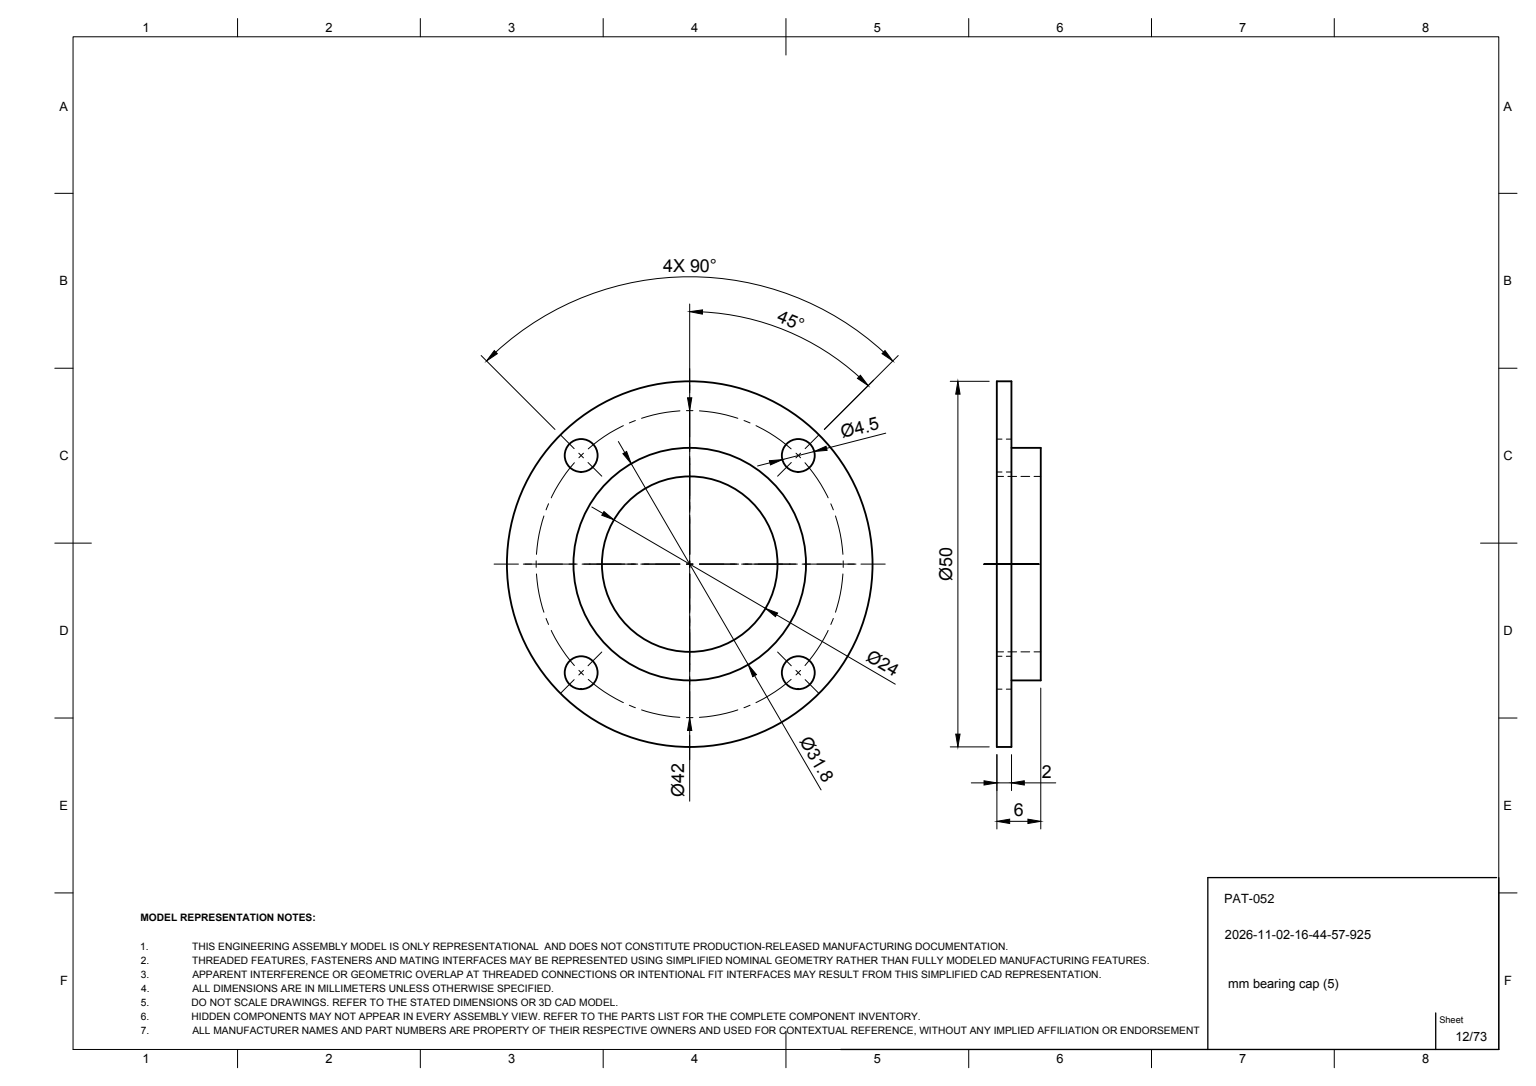
ISO-10303-21;
HEADER;
/* Generated by software containing ST-Developer
 * from STEP Tools, Inc. (www.steptools.com) 
 */

FILE_DESCRIPTION(
/* description */ ('Hand-crank gear train demonstrator'),
/* implementation_level */ '2;1');

FILE_NAME(
/* name */ 'mm bearing cap (5).step',
/* time_stamp */ '2026-10-28T03:22:13-07:00',
/* author */ (''),
/* organization */ (''),
/* preprocessor_version */ 'ST-DEVELOPER v20.2',
/* originating_system */ 'Autodesk Translation Framework v15.17.0.0',
/* authorisation */ '');

FILE_SCHEMA (('AUTOMOTIVE_DESIGN { 1 0 10303 214 3 1 1 }'));
ENDSEC;

DATA;
#10=MECHANICAL_DESIGN_GEOMETRIC_PRESENTATION_REPRESENTATION('',(#1197),#62758);
#1069=SHAPE_REPRESENTATION_RELATIONSHIP('SRR','None',#63041,#1133);
#1133=ADVANCED_BREP_SHAPE_REPRESENTATION('',(#1275),#62695);
#1197=STYLED_ITEM('',(#63462),#1275);
#1275=MANIFOLD_SOLID_BREP('Body1',#16378);
#1454=FACE_BOUND('',#3285,.T.);
#1455=FACE_BOUND('',#3289,.T.);
#1456=FACE_BOUND('',#3290,.T.);
#1457=FACE_BOUND('',#3291,.T.);
#1458=FACE_BOUND('',#3292,.T.);
#1459=FACE_BOUND('',#3293,.T.);
#1460=FACE_BOUND('',#3295,.T.);
#1461=FACE_BOUND('',#3296,.T.);
#1462=FACE_BOUND('',#3297,.T.);
#1463=FACE_BOUND('',#3298,.T.);
#1464=FACE_BOUND('',#3299,.T.);
#1673=PLANE('',#17425);
#1674=PLANE('',#17432);
#1675=PLANE('',#17433);
#2231=FACE_OUTER_BOUND('',#3279,.T.);
#2232=FACE_OUTER_BOUND('',#3280,.T.);
#2233=FACE_OUTER_BOUND('',#3281,.T.);
#2234=FACE_OUTER_BOUND('',#3282,.T.);
#2235=FACE_OUTER_BOUND('',#3283,.T.);
#2236=FACE_OUTER_BOUND('',#3284,.T.);
#2237=FACE_OUTER_BOUND('',#3286,.T.);
#2238=FACE_OUTER_BOUND('',#3287,.T.);
#2239=FACE_OUTER_BOUND('',#3288,.T.);
#2240=FACE_OUTER_BOUND('',#3294,.T.);
#3279=EDGE_LOOP('',(#11333,#11334,#11335,#11336));
#3280=EDGE_LOOP('',(#11337,#11338,#11339,#11340));
#3281=EDGE_LOOP('',(#11341,#11342,#11343,#11344));
#3282=EDGE_LOOP('',(#11345,#11346,#11347,#11348));
#3283=EDGE_LOOP('',(#11349,#11350,#11351,#11352));
#3284=EDGE_LOOP('',(#11353));
#3285=EDGE_LOOP('',(#11354));
#3286=EDGE_LOOP('',(#11355,#11356,#11357,#11358));
#3287=EDGE_LOOP('',(#11359,#11360,#11361,#11362));
#3288=EDGE_LOOP('',(#11363));
#3289=EDGE_LOOP('',(#11364));
#3290=EDGE_LOOP('',(#11365));
#3291=EDGE_LOOP('',(#11366));
#3292=EDGE_LOOP('',(#11367));
#3293=EDGE_LOOP('',(#11368));
#3294=EDGE_LOOP('',(#11369));
#3295=EDGE_LOOP('',(#11370));
#3296=EDGE_LOOP('',(#11371));
#3297=EDGE_LOOP('',(#11372));
#3298=EDGE_LOOP('',(#11373));
#3299=EDGE_LOOP('',(#11374));
#4402=LINE('',#23846,#5534);
#4403=LINE('',#23852,#5535);
#4404=LINE('',#23858,#5536);
#4405=LINE('',#23864,#5537);
#4406=LINE('',#23870,#5538);
#4407=LINE('',#23878,#5539);
#4408=LINE('',#23883,#5540);
#5534=VECTOR('',#19455,0.225);
#5535=VECTOR('',#19462,0.225);
#5536=VECTOR('',#19469,0.225);
#5537=VECTOR('',#19476,0.225);
#5538=VECTOR('',#19483,1.59);
#5539=VECTOR('',#19494,1.2);
#5540=VECTOR('',#19499,2.5);
#6683=CIRCLE('',#17411,0.225);
#6684=CIRCLE('',#17412,0.225);
#6685=CIRCLE('',#17414,0.225);
#6686=CIRCLE('',#17415,0.225);
#6687=CIRCLE('',#17417,0.225);
#6688=CIRCLE('',#17418,0.225);
#6689=CIRCLE('',#17420,0.225);
#6690=CIRCLE('',#17421,0.225);
#6691=CIRCLE('',#17423,1.59);
#6692=CIRCLE('',#17424,1.59);
#6693=CIRCLE('',#17426,1.2);
#6694=CIRCLE('',#17428,1.2);
#6695=CIRCLE('',#17430,2.5);
#6696=CIRCLE('',#17431,2.5);
#7377=VERTEX_POINT('',#23843);
#7378=VERTEX_POINT('',#23845);
#7379=VERTEX_POINT('',#23849);
#7380=VERTEX_POINT('',#23851);
#7381=VERTEX_POINT('',#23855);
#7382=VERTEX_POINT('',#23857);
#7383=VERTEX_POINT('',#23861);
#7384=VERTEX_POINT('',#23863);
#7385=VERTEX_POINT('',#23867);
#7386=VERTEX_POINT('',#23869);
#7387=VERTEX_POINT('',#23873);
#7388=VERTEX_POINT('',#23876);
#7389=VERTEX_POINT('',#23880);
#7390=VERTEX_POINT('',#23882);
#8918=EDGE_CURVE('',#7377,#7377,#6683,.T.);
#8919=EDGE_CURVE('',#7377,#7378,#4402,.T.);
#8920=EDGE_CURVE('',#7378,#7378,#6684,.T.);
#8921=EDGE_CURVE('',#7379,#7379,#6685,.T.);
#8922=EDGE_CURVE('',#7379,#7380,#4403,.T.);
#8923=EDGE_CURVE('',#7380,#7380,#6686,.T.);
#8924=EDGE_CURVE('',#7381,#7381,#6687,.T.);
#8925=EDGE_CURVE('',#7381,#7382,#4404,.T.);
#8926=EDGE_CURVE('',#7382,#7382,#6688,.T.);
#8927=EDGE_CURVE('',#7383,#7383,#6689,.T.);
#8928=EDGE_CURVE('',#7383,#7384,#4405,.T.);
#8929=EDGE_CURVE('',#7384,#7384,#6690,.T.);
#8930=EDGE_CURVE('',#7385,#7385,#6691,.T.);
#8931=EDGE_CURVE('',#7385,#7386,#4406,.T.);
#8932=EDGE_CURVE('',#7386,#7386,#6692,.T.);
#8933=EDGE_CURVE('',#7387,#7387,#6693,.T.);
#8934=EDGE_CURVE('',#7388,#7388,#6694,.T.);
#8935=EDGE_CURVE('',#7388,#7387,#4407,.T.);
#8936=EDGE_CURVE('',#7389,#7389,#6695,.T.);
#8937=EDGE_CURVE('',#7389,#7390,#4408,.T.);
#8938=EDGE_CURVE('',#7390,#7390,#6696,.T.);
#11333=ORIENTED_EDGE('',*,*,#8918,.F.);
#11334=ORIENTED_EDGE('',*,*,#8919,.T.);
#11335=ORIENTED_EDGE('',*,*,#8920,.F.);
#11336=ORIENTED_EDGE('',*,*,#8919,.F.);
#11337=ORIENTED_EDGE('',*,*,#8921,.F.);
#11338=ORIENTED_EDGE('',*,*,#8922,.T.);
#11339=ORIENTED_EDGE('',*,*,#8923,.F.);
#11340=ORIENTED_EDGE('',*,*,#8922,.F.);
#11341=ORIENTED_EDGE('',*,*,#8924,.F.);
#11342=ORIENTED_EDGE('',*,*,#8925,.T.);
#11343=ORIENTED_EDGE('',*,*,#8926,.F.);
#11344=ORIENTED_EDGE('',*,*,#8925,.F.);
#11345=ORIENTED_EDGE('',*,*,#8927,.F.);
#11346=ORIENTED_EDGE('',*,*,#8928,.T.);
#11347=ORIENTED_EDGE('',*,*,#8929,.F.);
#11348=ORIENTED_EDGE('',*,*,#8928,.F.);
#11349=ORIENTED_EDGE('',*,*,#8930,.F.);
#11350=ORIENTED_EDGE('',*,*,#8931,.T.);
#11351=ORIENTED_EDGE('',*,*,#8932,.T.);
#11352=ORIENTED_EDGE('',*,*,#8931,.F.);
#11353=ORIENTED_EDGE('',*,*,#8932,.F.);
#11354=ORIENTED_EDGE('',*,*,#8933,.F.);
#11355=ORIENTED_EDGE('',*,*,#8934,.F.);
#11356=ORIENTED_EDGE('',*,*,#8935,.T.);
#11357=ORIENTED_EDGE('',*,*,#8933,.T.);
#11358=ORIENTED_EDGE('',*,*,#8935,.F.);
#11359=ORIENTED_EDGE('',*,*,#8936,.F.);
#11360=ORIENTED_EDGE('',*,*,#8937,.T.);
#11361=ORIENTED_EDGE('',*,*,#8938,.T.);
#11362=ORIENTED_EDGE('',*,*,#8937,.F.);
#11363=ORIENTED_EDGE('',*,*,#8936,.T.);
#11364=ORIENTED_EDGE('',*,*,#8934,.T.);
#11365=ORIENTED_EDGE('',*,*,#8929,.T.);
#11366=ORIENTED_EDGE('',*,*,#8926,.T.);
#11367=ORIENTED_EDGE('',*,*,#8923,.T.);
#11368=ORIENTED_EDGE('',*,*,#8920,.T.);
#11369=ORIENTED_EDGE('',*,*,#8938,.F.);
#11370=ORIENTED_EDGE('',*,*,#8930,.T.);
#11371=ORIENTED_EDGE('',*,*,#8927,.T.);
#11372=ORIENTED_EDGE('',*,*,#8924,.T.);
#11373=ORIENTED_EDGE('',*,*,#8921,.T.);
#11374=ORIENTED_EDGE('',*,*,#8918,.T.);
#15232=CYLINDRICAL_SURFACE('',#17410,0.225);
#15233=CYLINDRICAL_SURFACE('',#17413,0.225);
#15234=CYLINDRICAL_SURFACE('',#17416,0.225);
#15235=CYLINDRICAL_SURFACE('',#17419,0.225);
#15236=CYLINDRICAL_SURFACE('',#17422,1.59);
#15237=CYLINDRICAL_SURFACE('',#17427,1.2);
#15238=CYLINDRICAL_SURFACE('',#17429,2.5);
#15541=ADVANCED_FACE('',(#2231),#15232,.F.);
#15542=ADVANCED_FACE('',(#2232),#15233,.F.);
#15543=ADVANCED_FACE('',(#2233),#15234,.F.);
#15544=ADVANCED_FACE('',(#2234),#15235,.F.);
#15545=ADVANCED_FACE('',(#2235),#15236,.T.);
#15546=ADVANCED_FACE('',(#2236,#1454),#1673,.F.);
#15547=ADVANCED_FACE('',(#2237),#15237,.F.);
#15548=ADVANCED_FACE('',(#2238),#15238,.T.);
#15549=ADVANCED_FACE('',(#2239,#1455,#1456,#1457,#1458,#1459),#1674,.T.);
#15550=ADVANCED_FACE('',(#2240,#1460,#1461,#1462,#1463,#1464),#1675,.F.);
#16378=CLOSED_SHELL('',(#15541,#15542,#15543,#15544,#15545,#15546,#15547,
#15548,#15549,#15550));
#17409=AXIS2_PLACEMENT_3D('',#23841,#19449,#19450);
#17410=AXIS2_PLACEMENT_3D('',#23842,#19451,#19452);
#17411=AXIS2_PLACEMENT_3D('',#23844,#19453,#19454);
#17412=AXIS2_PLACEMENT_3D('',#23847,#19456,#19457);
#17413=AXIS2_PLACEMENT_3D('',#23848,#19458,#19459);
#17414=AXIS2_PLACEMENT_3D('',#23850,#19460,#19461);
#17415=AXIS2_PLACEMENT_3D('',#23853,#19463,#19464);
#17416=AXIS2_PLACEMENT_3D('',#23854,#19465,#19466);
#17417=AXIS2_PLACEMENT_3D('',#23856,#19467,#19468);
#17418=AXIS2_PLACEMENT_3D('',#23859,#19470,#19471);
#17419=AXIS2_PLACEMENT_3D('',#23860,#19472,#19473);
#17420=AXIS2_PLACEMENT_3D('',#23862,#19474,#19475);
#17421=AXIS2_PLACEMENT_3D('',#23865,#19477,#19478);
#17422=AXIS2_PLACEMENT_3D('',#23866,#19479,#19480);
#17423=AXIS2_PLACEMENT_3D('',#23868,#19481,#19482);
#17424=AXIS2_PLACEMENT_3D('',#23871,#19484,#19485);
#17425=AXIS2_PLACEMENT_3D('',#23872,#19486,#19487);
#17426=AXIS2_PLACEMENT_3D('',#23874,#19488,#19489);
#17427=AXIS2_PLACEMENT_3D('',#23875,#19490,#19491);
#17428=AXIS2_PLACEMENT_3D('',#23877,#19492,#19493);
#17429=AXIS2_PLACEMENT_3D('',#23879,#19495,#19496);
#17430=AXIS2_PLACEMENT_3D('',#23881,#19497,#19498);
#17431=AXIS2_PLACEMENT_3D('',#23884,#19500,#19501);
#17432=AXIS2_PLACEMENT_3D('',#23885,#19502,#19503);
#17433=AXIS2_PLACEMENT_3D('',#23886,#19504,#19505);
#19449=DIRECTION('axis',(0.,0.,1.));
#19450=DIRECTION('refdir',(1.,0.,0.));
#19451=DIRECTION('center_axis',(0.,1.,0.));
#19452=DIRECTION('ref_axis',(1.,0.,0.));
#19453=DIRECTION('center_axis',(0.,1.,0.));
#19454=DIRECTION('ref_axis',(1.,0.,0.));
#19455=DIRECTION('',(0.,1.,0.));
#19456=DIRECTION('center_axis',(0.,-1.,0.));
#19457=DIRECTION('ref_axis',(1.,0.,0.));
#19458=DIRECTION('center_axis',(0.,1.,0.));
#19459=DIRECTION('ref_axis',(1.,0.,0.));
#19460=DIRECTION('center_axis',(0.,1.,0.));
#19461=DIRECTION('ref_axis',(1.,0.,0.));
#19462=DIRECTION('',(0.,1.,0.));
#19463=DIRECTION('center_axis',(0.,-1.,0.));
#19464=DIRECTION('ref_axis',(1.,0.,0.));
#19465=DIRECTION('center_axis',(0.,1.,0.));
#19466=DIRECTION('ref_axis',(1.,0.,0.));
#19467=DIRECTION('center_axis',(0.,1.,0.));
#19468=DIRECTION('ref_axis',(1.,0.,0.));
#19469=DIRECTION('',(0.,1.,0.));
#19470=DIRECTION('center_axis',(0.,-1.,0.));
#19471=DIRECTION('ref_axis',(1.,0.,0.));
#19472=DIRECTION('center_axis',(0.,1.,0.));
#19473=DIRECTION('ref_axis',(1.,0.,0.));
#19474=DIRECTION('center_axis',(0.,1.,0.));
#19475=DIRECTION('ref_axis',(1.,0.,0.));
#19476=DIRECTION('',(0.,1.,0.));
#19477=DIRECTION('center_axis',(0.,-1.,0.));
#19478=DIRECTION('ref_axis',(1.,0.,0.));
#19479=DIRECTION('center_axis',(0.,1.,0.));
#19480=DIRECTION('ref_axis',(1.,0.,0.));
#19481=DIRECTION('center_axis',(0.,1.,0.));
#19482=DIRECTION('ref_axis',(1.,0.,0.));
#19483=DIRECTION('',(0.,-1.,0.));
#19484=DIRECTION('center_axis',(0.,1.,0.));
#19485=DIRECTION('ref_axis',(1.,0.,0.));
#19486=DIRECTION('center_axis',(0.,1.,0.));
#19487=DIRECTION('ref_axis',(1.,0.,0.));
#19488=DIRECTION('center_axis',(0.,-1.,0.));
#19489=DIRECTION('ref_axis',(1.,0.,0.));
#19490=DIRECTION('center_axis',(0.,1.,0.));
#19491=DIRECTION('ref_axis',(1.,0.,0.));
#19492=DIRECTION('center_axis',(0.,-1.,0.));
#19493=DIRECTION('ref_axis',(1.,0.,0.));
#19494=DIRECTION('',(0.,-1.,0.));
#19495=DIRECTION('center_axis',(0.,1.,0.));
#19496=DIRECTION('ref_axis',(1.,0.,0.));
#19497=DIRECTION('center_axis',(0.,1.,0.));
#19498=DIRECTION('ref_axis',(1.,0.,0.));
#19499=DIRECTION('',(0.,-1.,0.));
#19500=DIRECTION('center_axis',(0.,1.,0.));
#19501=DIRECTION('ref_axis',(1.,0.,0.));
#19502=DIRECTION('center_axis',(0.,1.,0.));
#19503=DIRECTION('ref_axis',(1.,0.,0.));
#19504=DIRECTION('center_axis',(0.,1.,0.));
#19505=DIRECTION('ref_axis',(1.,0.,0.));
#23841=CARTESIAN_POINT('',(0.,0.,0.));
#23842=CARTESIAN_POINT('Origin',(10.5150757595082,-0.7,7.51507575950825));
#23843=CARTESIAN_POINT('',(10.2900757595082,-0.6,7.51507575950825));
#23844=CARTESIAN_POINT('Origin',(10.5150757595082,-0.6,7.51507575950825));
#23845=CARTESIAN_POINT('',(10.2900757595082,-0.4,7.51507575950825));
#23846=CARTESIAN_POINT('',(10.2900757595082,-0.7,7.51507575950825));
#23847=CARTESIAN_POINT('Origin',(10.5150757595082,-0.4,7.51507575950825));
#23848=CARTESIAN_POINT('Origin',(10.5150757595082,-0.7,10.4849242404918));
#23849=CARTESIAN_POINT('',(10.2900757595082,-0.6,10.4849242404918));
#23850=CARTESIAN_POINT('Origin',(10.5150757595082,-0.6,10.4849242404918));
#23851=CARTESIAN_POINT('',(10.2900757595082,-0.4,10.4849242404918));
#23852=CARTESIAN_POINT('',(10.2900757595082,-0.7,10.4849242404918));
#23853=CARTESIAN_POINT('Origin',(10.5150757595082,-0.4,10.4849242404918));
#23854=CARTESIAN_POINT('Origin',(13.4849242404918,-0.7,10.4849242404918));
#23855=CARTESIAN_POINT('',(13.2599242404918,-0.6,10.4849242404918));
#23856=CARTESIAN_POINT('Origin',(13.4849242404918,-0.6,10.4849242404918));
#23857=CARTESIAN_POINT('',(13.2599242404918,-0.4,10.4849242404918));
#23858=CARTESIAN_POINT('',(13.2599242404918,-0.7,10.4849242404918));
#23859=CARTESIAN_POINT('Origin',(13.4849242404918,-0.4,10.4849242404918));
#23860=CARTESIAN_POINT('Origin',(13.4849242404918,-0.7,7.51507575950825));
#23861=CARTESIAN_POINT('',(13.2599242404918,-0.6,7.51507575950825));
#23862=CARTESIAN_POINT('Origin',(13.4849242404918,-0.6,7.51507575950825));
#23863=CARTESIAN_POINT('',(13.2599242404918,-0.4,7.51507575950825));
#23864=CARTESIAN_POINT('',(13.2599242404918,-0.7,7.51507575950825));
#23865=CARTESIAN_POINT('Origin',(13.4849242404918,-0.4,7.51507575950825));
#23866=CARTESIAN_POINT('Origin',(12.,-1.,9.));
#23867=CARTESIAN_POINT('',(10.41,-0.6,9.));
#23868=CARTESIAN_POINT('Origin',(12.,-0.6,9.));
#23869=CARTESIAN_POINT('',(10.41,-1.,9.));
#23870=CARTESIAN_POINT('',(10.41,-1.,9.));
#23871=CARTESIAN_POINT('Origin',(12.,-1.,9.));
#23872=CARTESIAN_POINT('Origin',(12.,-1.,9.));
#23873=CARTESIAN_POINT('',(10.8,-1.,9.));
#23874=CARTESIAN_POINT('Origin',(12.,-1.,9.));
#23875=CARTESIAN_POINT('Origin',(12.,-0.6,9.));
#23876=CARTESIAN_POINT('',(10.8,-0.4,9.));
#23877=CARTESIAN_POINT('Origin',(12.,-0.4,9.));
#23878=CARTESIAN_POINT('',(10.8,-0.6,9.));
#23879=CARTESIAN_POINT('Origin',(12.,-0.6,9.));
#23880=CARTESIAN_POINT('',(9.5,-0.4,9.));
#23881=CARTESIAN_POINT('Origin',(12.,-0.4,9.));
#23882=CARTESIAN_POINT('',(9.5,-0.6,9.));
#23883=CARTESIAN_POINT('',(9.5,-0.6,9.));
#23884=CARTESIAN_POINT('Origin',(12.,-0.6,9.));
#23885=CARTESIAN_POINT('Origin',(12.,-0.4,9.));
#23886=CARTESIAN_POINT('Origin',(12.,-0.6,9.));
#62621=UNCERTAINTY_MEASURE_WITH_UNIT(LENGTH_MEASURE(0.001),#62759,
'DISTANCE_ACCURACY_VALUE',
'Maximum model space distance between geometric entities at asserted c
onnectivities');
#62684=UNCERTAINTY_MEASURE_WITH_UNIT(LENGTH_MEASURE(0.001),#62759,
'DISTANCE_ACCURACY_VALUE',
'Maximum model space distance between geometric entities at asserted c
onnectivities');
#62695=(
GEOMETRIC_REPRESENTATION_CONTEXT(3)
GLOBAL_UNCERTAINTY_ASSIGNED_CONTEXT((#62621))
GLOBAL_UNIT_ASSIGNED_CONTEXT((#62759,#62761,#62762))
REPRESENTATION_CONTEXT('','3D')
);
#62758=(
GEOMETRIC_REPRESENTATION_CONTEXT(3)
GLOBAL_UNCERTAINTY_ASSIGNED_CONTEXT((#62684))
GLOBAL_UNIT_ASSIGNED_CONTEXT((#62759,#62761,#62762))
REPRESENTATION_CONTEXT('','3D')
);
#62759=(
LENGTH_UNIT()
NAMED_UNIT(*)
SI_UNIT(.CENTI.,.METRE.)
);
#62761=(
NAMED_UNIT(*)
PLANE_ANGLE_UNIT()
SI_UNIT($,.RADIAN.)
);
#62762=(
NAMED_UNIT(*)
SI_UNIT($,.STERADIAN.)
SOLID_ANGLE_UNIT()
);
#62773=SHAPE_DEFINITION_REPRESENTATION(#62846,#63041);
#62846=PRODUCT_DEFINITION_SHAPE('',$,#63115);
#63041=SHAPE_REPRESENTATION('',(#17409),#62695);
#63104=PRODUCT_DEFINITION_CONTEXT('part definition',#63325,'design');
#63115=PRODUCT_DEFINITION('mm bearing cap (5)','mm bearing cap (5)',#63188,
#63104);
#63188=PRODUCT_DEFINITION_FORMATION('',$,#63337);
#63325=APPLICATION_CONTEXT(
'Core Data for Automotive Mechanical Design Process');
#63326=PRODUCT_CONTEXT('part definition',#63325,'mechanical');
#63337=PRODUCT('mm bearing cap (5)','mm bearing cap (5)','mm bearing cap (5)',
(#63326));
#63456=COLOUR_RGB('Grey',0.48,0.52,0.57);
#63457=FILL_AREA_STYLE_COLOUR('',#63456);
#63458=FILL_AREA_STYLE('',(#63457));
#63459=SURFACE_STYLE_FILL_AREA(#63458);
#63460=SURFACE_SIDE_STYLE('',(#63459));
#63461=SURFACE_STYLE_USAGE(.BOTH.,#63460);
#63462=PRESENTATION_STYLE_ASSIGNMENT((#63461));
ENDSEC;
END-ISO-10303-21;
